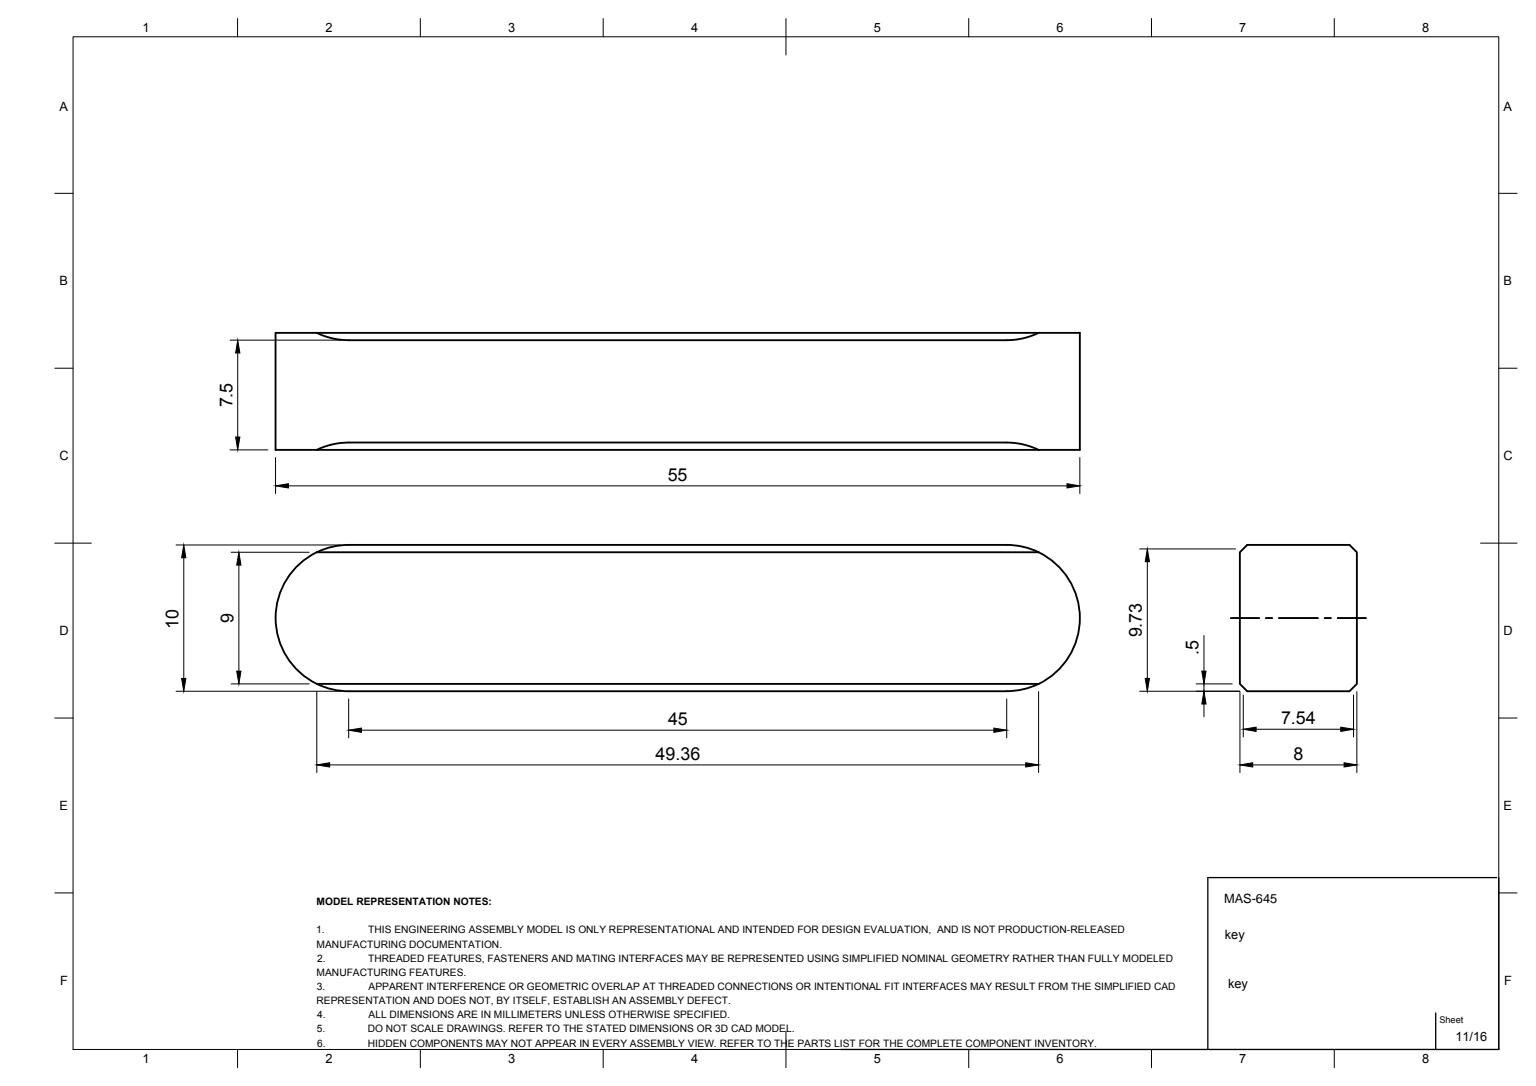
ISO-10303-21;
HEADER;
FILE_DESCRIPTION((''),'2;1');
FILE_NAME('Key.step','2026-10-09T10:54:55-07:00',(''),(''),'','','');
FILE_SCHEMA (('AUTOMOTIVE_DESIGN { 1 0 10303 214 3 1 1 }'));
ENDSEC;
DATA;
#10=MECHANICAL_DESIGN_GEOMETRIC_PRESENTATION_REPRESENTATION('',(#601),#63824);
#91=ELLIPSE('',#16171,7.07106781186547,5.) ;
#92=ELLIPSE('',#16172,7.07106781186548,5.) ;
#93=ELLIPSE('',#16174,7.07106781186548,5.) ;
#94=ELLIPSE('',#16175,7.07106781186547,5.) ;
#95=ELLIPSE('',#16178,7.07106781186546,4.99999999999999) ;
#96=ELLIPSE('',#16180,7.07106781186546,4.99999999999999) ;
#97=ELLIPSE('',#16181,7.07106781186546,4.99999999999999) ;
#98=ELLIPSE('',#16183,7.07106781186546,4.99999999999999) ;
#571=SHAPE_REPRESENTATION_RELATIONSHIP('SRR','None',#63885,#586) ;
#586=ADVANCED_BREP_SHAPE_REPRESENTATION('',(#616),#63815) ;
#601=STYLED_ITEM('',(#63963),#616) ;
#616=MANIFOLD_SOLID_BREP('Body1',#15500) ;
#898=PLANE('',#16176) ;
#899=PLANE('',#16184) ;
#900=PLANE('',#16185) ;
#901=PLANE('',#16186) ;
#902=PLANE('',#16187) ;
#903=PLANE('',#16188) ;
#904=PLANE('',#16189) ;
#905=PLANE('',#16190) ;
#1260=CYLINDRICAL_SURFACE('',#16169,5.) ;
#1261=CYLINDRICAL_SURFACE('',#16177,4.99999999999999) ;
#1815=FACE_OUTER_BOUND('',#2799,.T.) ;
#1816=FACE_OUTER_BOUND('',#2800,.T.) ;
#1817=FACE_OUTER_BOUND('',#2801,.T.) ;
#1818=FACE_OUTER_BOUND('',#2802,.T.) ;
#1819=FACE_OUTER_BOUND('',#2803,.T.) ;
#1820=FACE_OUTER_BOUND('',#2804,.T.) ;
#1821=FACE_OUTER_BOUND('',#2805,.T.) ;
#1822=FACE_OUTER_BOUND('',#2806,.T.) ;
#1823=FACE_OUTER_BOUND('',#2807,.T.) ;
#1824=FACE_OUTER_BOUND('',#2808,.T.) ;
#2799=EDGE_LOOP('',(#10982,#10983,#10984,#10985,#10986,#10987,#10988,#10989)) ;
#2800=EDGE_LOOP('',(#10990,#10991,#10992,#10993)) ;
#2801=EDGE_LOOP('',(#10994,#10995,#10996,#10997,#10998,#10999,#11000,#11001)) ;
#2802=EDGE_LOOP('',(#11002,#11003,#11004,#11005)) ;
#2803=EDGE_LOOP('',(#11006,#11007,#11008,#11009)) ;
#2804=EDGE_LOOP('',(#11010,#11011,#11012,#11013)) ;
#2805=EDGE_LOOP('',(#11014,#11015,#11016,#11017)) ;
#2806=EDGE_LOOP('',(#11018,#11019,#11020,#11021)) ;
#2807=EDGE_LOOP('',(#11022,#11023,#11024,#11025)) ;
#2808=EDGE_LOOP('',(#11026,#11027,#11028,#11029)) ;
#3697=CIRCLE('',#16170,5.) ;
#3698=CIRCLE('',#16173,5.) ;
#3699=CIRCLE('',#16179,4.99999999999999) ;
#3700=CIRCLE('',#16182,4.99999999999999) ;
#4946=LINE('',#51875,#5602) ;
#4947=LINE('',#51883,#5603) ;
#4948=LINE('',#51887,#5604) ;
#4949=LINE('',#51889,#5605) ;
#4950=LINE('',#51890,#5606) ;
#4951=LINE('',#51894,#5607) ;
#4952=LINE('',#51906,#5608) ;
#4953=LINE('',#51907,#5609) ;
#4954=LINE('',#51909,#5610) ;
#4955=LINE('',#51910,#5611) ;
#4956=LINE('',#51912,#5612) ;
#4957=LINE('',#51913,#5613) ;
#5602=VECTOR('',#19152,1000.) ;
#5603=VECTOR('',#19159,1000.) ;
#5604=VECTOR('',#19164,1000.) ;
#5605=VECTOR('',#19165,1000.) ;
#5606=VECTOR('',#19166,1000.) ;
#5607=VECTOR('',#19169,1000.) ;
#5608=VECTOR('',#19184,1000.) ;
#5609=VECTOR('',#19185,1000.) ;
#5610=VECTOR('',#19188,1000.) ;
#5611=VECTOR('',#19189,1000.) ;
#5612=VECTOR('',#19192,1000.) ;
#5613=VECTOR('',#19193,1000.) ;
#6411=VERTEX_POINT('',#51869) ;
#6412=VERTEX_POINT('',#51870) ;
#6413=VERTEX_POINT('',#51872) ;
#6414=VERTEX_POINT('',#51874) ;
#6415=VERTEX_POINT('',#51876) ;
#6416=VERTEX_POINT('',#51878) ;
#6417=VERTEX_POINT('',#51880) ;
#6418=VERTEX_POINT('',#51882) ;
#6419=VERTEX_POINT('',#51886) ;
#6420=VERTEX_POINT('',#51888) ;
#6421=VERTEX_POINT('',#51892) ;
#6422=VERTEX_POINT('',#51893) ;
#6423=VERTEX_POINT('',#51895) ;
#6424=VERTEX_POINT('',#51897) ;
#6425=VERTEX_POINT('',#51900) ;
#6426=VERTEX_POINT('',#51902) ;
#8045=EDGE_CURVE('',#6411,#6412,#3697,.T.) ;
#8046=EDGE_CURVE('',#6412,#6413,#91,.T.) ;
#8047=EDGE_CURVE('',#6414,#6413,#4946,.T.) ;
#8048=EDGE_CURVE('',#6414,#6415,#92,.T.) ;
#8049=EDGE_CURVE('',#6416,#6415,#3698,.T.) ;
#8050=EDGE_CURVE('',#6416,#6417,#93,.T.) ;
#8051=EDGE_CURVE('',#6417,#6418,#4947,.T.) ;
#8052=EDGE_CURVE('',#6418,#6411,#94,.T.) ;
#8053=EDGE_CURVE('',#6419,#6413,#4948,.T.) ;
#8054=EDGE_CURVE('',#6420,#6419,#4949,.T.) ;
#8055=EDGE_CURVE('',#6420,#6414,#4950,.T.) ;
#8056=EDGE_CURVE('',#6421,#6422,#4951,.T.) ;
#8057=EDGE_CURVE('',#6421,#6423,#95,.T.) ;
#8058=EDGE_CURVE('',#6424,#6423,#3699,.T.) ;
#8059=EDGE_CURVE('',#6424,#6420,#96,.T.) ;
#8060=EDGE_CURVE('',#6419,#6425,#97,.T.) ;
#8061=EDGE_CURVE('',#6425,#6426,#3700,.T.) ;
#8062=EDGE_CURVE('',#6426,#6422,#98,.T.) ;
#8063=EDGE_CURVE('',#6421,#6417,#4952,.T.) ;
#8064=EDGE_CURVE('',#6422,#6418,#4953,.T.) ;
#8065=EDGE_CURVE('',#6416,#6423,#4954,.T.) ;
#8066=EDGE_CURVE('',#6424,#6415,#4955,.T.) ;
#8067=EDGE_CURVE('',#6411,#6426,#4956,.T.) ;
#8068=EDGE_CURVE('',#6425,#6412,#4957,.T.) ;
#10982=ORIENTED_EDGE('',*,*,#8045,.T.) ;
#10983=ORIENTED_EDGE('',*,*,#8046,.T.) ;
#10984=ORIENTED_EDGE('',*,*,#8047,.F.) ;
#10985=ORIENTED_EDGE('',*,*,#8048,.T.) ;
#10986=ORIENTED_EDGE('',*,*,#8049,.F.) ;
#10987=ORIENTED_EDGE('',*,*,#8050,.T.) ;
#10988=ORIENTED_EDGE('',*,*,#8051,.T.) ;
#10989=ORIENTED_EDGE('',*,*,#8052,.T.) ;
#10990=ORIENTED_EDGE('',*,*,#8047,.T.) ;
#10991=ORIENTED_EDGE('',*,*,#8053,.F.) ;
#10992=ORIENTED_EDGE('',*,*,#8054,.F.) ;
#10993=ORIENTED_EDGE('',*,*,#8055,.T.) ;
#10994=ORIENTED_EDGE('',*,*,#8056,.F.) ;
#10995=ORIENTED_EDGE('',*,*,#8057,.T.) ;
#10996=ORIENTED_EDGE('',*,*,#8058,.F.) ;
#10997=ORIENTED_EDGE('',*,*,#8059,.T.) ;
#10998=ORIENTED_EDGE('',*,*,#8054,.T.) ;
#10999=ORIENTED_EDGE('',*,*,#8060,.T.) ;
#11000=ORIENTED_EDGE('',*,*,#8061,.T.) ;
#11001=ORIENTED_EDGE('',*,*,#8062,.T.) ;
#11002=ORIENTED_EDGE('',*,*,#8051,.F.) ;
#11003=ORIENTED_EDGE('',*,*,#8063,.F.) ;
#11004=ORIENTED_EDGE('',*,*,#8056,.T.) ;
#11005=ORIENTED_EDGE('',*,*,#8064,.T.) ;
#11006=ORIENTED_EDGE('',*,*,#8065,.F.) ;
#11007=ORIENTED_EDGE('',*,*,#8049,.T.) ;
#11008=ORIENTED_EDGE('',*,*,#8066,.F.) ;
#11009=ORIENTED_EDGE('',*,*,#8058,.T.) ;
#11010=ORIENTED_EDGE('',*,*,#8045,.F.) ;
#11011=ORIENTED_EDGE('',*,*,#8067,.T.) ;
#11012=ORIENTED_EDGE('',*,*,#8061,.F.) ;
#11013=ORIENTED_EDGE('',*,*,#8068,.T.) ;
#11014=ORIENTED_EDGE('',*,*,#8068,.F.) ;
#11015=ORIENTED_EDGE('',*,*,#8060,.F.) ;
#11016=ORIENTED_EDGE('',*,*,#8053,.T.) ;
#11017=ORIENTED_EDGE('',*,*,#8046,.F.) ;
#11018=ORIENTED_EDGE('',*,*,#8064,.F.) ;
#11019=ORIENTED_EDGE('',*,*,#8062,.F.) ;
#11020=ORIENTED_EDGE('',*,*,#8067,.F.) ;
#11021=ORIENTED_EDGE('',*,*,#8052,.F.) ;
#11022=ORIENTED_EDGE('',*,*,#8055,.F.) ;
#11023=ORIENTED_EDGE('',*,*,#8059,.F.) ;
#11024=ORIENTED_EDGE('',*,*,#8066,.T.) ;
#11025=ORIENTED_EDGE('',*,*,#8048,.F.) ;
#11026=ORIENTED_EDGE('',*,*,#8065,.T.) ;
#11027=ORIENTED_EDGE('',*,*,#8057,.F.) ;
#11028=ORIENTED_EDGE('',*,*,#8063,.T.) ;
#11029=ORIENTED_EDGE('',*,*,#8050,.F.) ;
#14903=ADVANCED_FACE('',(#1815),#1260,.T.) ;
#14904=ADVANCED_FACE('',(#1816),#898,.F.) ;
#14905=ADVANCED_FACE('',(#1817),#1261,.T.) ;
#14906=ADVANCED_FACE('',(#1818),#899,.F.) ;
#14907=ADVANCED_FACE('',(#1819),#900,.T.) ;
#14908=ADVANCED_FACE('',(#1820),#901,.F.) ;
#14909=ADVANCED_FACE('',(#1821),#902,.F.) ;
#14910=ADVANCED_FACE('',(#1822),#903,.F.) ;
#14911=ADVANCED_FACE('',(#1823),#904,.F.) ;
#14912=ADVANCED_FACE('',(#1824),#905,.F.) ;
#15500=CLOSED_SHELL('',(#14903,#14904,#14905,#14906,#14907,#14908,#14909,
#14910,#14911,#14912)) ;
#16168=AXIS2_PLACEMENT_3D('',#51867,#19144,#19145) ;
#16169=AXIS2_PLACEMENT_3D('',#51868,#19146,#19147) ;
#16170=AXIS2_PLACEMENT_3D('',#51871,#19148,#19149) ;
#16171=AXIS2_PLACEMENT_3D('',#51873,#19150,#19151) ;
#16172=AXIS2_PLACEMENT_3D('',#51877,#19153,#19154) ;
#16173=AXIS2_PLACEMENT_3D('',#51879,#19155,#19156) ;
#16174=AXIS2_PLACEMENT_3D('',#51881,#19157,#19158) ;
#16175=AXIS2_PLACEMENT_3D('',#51884,#19160,#19161) ;
#16176=AXIS2_PLACEMENT_3D('',#51885,#19162,#19163) ;
#16177=AXIS2_PLACEMENT_3D('',#51891,#19167,#19168) ;
#16178=AXIS2_PLACEMENT_3D('',#51896,#19170,#19171) ;
#16179=AXIS2_PLACEMENT_3D('',#51898,#19172,#19173) ;
#16180=AXIS2_PLACEMENT_3D('',#51899,#19174,#19175) ;
#16181=AXIS2_PLACEMENT_3D('',#51901,#19176,#19177) ;
#16182=AXIS2_PLACEMENT_3D('',#51903,#19178,#19179) ;
#16183=AXIS2_PLACEMENT_3D('',#51904,#19180,#19181) ;
#16184=AXIS2_PLACEMENT_3D('',#51905,#19182,#19183) ;
#16185=AXIS2_PLACEMENT_3D('',#51908,#19186,#19187) ;
#16186=AXIS2_PLACEMENT_3D('',#51911,#19190,#19191) ;
#16187=AXIS2_PLACEMENT_3D('',#51914,#19194,#19195) ;
#16188=AXIS2_PLACEMENT_3D('',#51915,#19196,#19197) ;
#16189=AXIS2_PLACEMENT_3D('',#51916,#19198,#19199) ;
#16190=AXIS2_PLACEMENT_3D('',#51917,#19200,#19201) ;
#19144=DIRECTION('axis',(0.,0.,1.)) ;
#19145=DIRECTION('refdir',(1.,0.,0.)) ;
#19146=DIRECTION('center_axis',(0.,0.,-1.)) ;
#19147=DIRECTION('ref_axis',(-1.,0.,0.)) ;
#19148=DIRECTION('center_axis',(0.,0.,1.)) ;
#19149=DIRECTION('ref_axis',(1.,0.,0.)) ;
#19150=DIRECTION('center_axis',(0.,0.707106781186548,0.707106781186548)) ;
#19151=DIRECTION('ref_axis',(0.,0.707106781186548,-0.707106781186548)) ;
#19152=DIRECTION('',(0.,0.,-1.)) ;
#19153=DIRECTION('center_axis',(0.,0.707106781186548,-0.707106781186547)) ;
#19154=DIRECTION('ref_axis',(0.,-0.707106781186547,-0.707106781186548)) ;
#19155=DIRECTION('center_axis',(0.,0.,1.)) ;
#19156=DIRECTION('ref_axis',(1.,0.,0.)) ;
#19157=DIRECTION('center_axis',(0.,-0.707106781186548,-0.707106781186548)) ;
#19158=DIRECTION('ref_axis',(0.,0.707106781186548,-0.707106781186548)) ;
#19159=DIRECTION('',(0.,0.,-1.)) ;
#19160=DIRECTION('center_axis',(0.,-0.707106781186547,0.707106781186548)) ;
#19161=DIRECTION('ref_axis',(0.,-0.707106781186548,-0.707106781186547)) ;
#19162=DIRECTION('center_axis',(0.,1.,0.)) ;
#19163=DIRECTION('ref_axis',(0.,0.,1.)) ;
#19164=DIRECTION('',(-1.,0.,0.)) ;
#19165=DIRECTION('',(0.,0.,-1.)) ;
#19166=DIRECTION('',(-1.,0.,0.)) ;
#19167=DIRECTION('center_axis',(0.,0.,-1.)) ;
#19168=DIRECTION('ref_axis',(1.,1.22464679914735E-16,0.)) ;
#19169=DIRECTION('',(0.,0.,-1.)) ;
#19170=DIRECTION('center_axis',(0.,-0.707106781186548,-0.707106781186548)) ;
#19171=DIRECTION('ref_axis',(0.,0.707106781186548,-0.707106781186548)) ;
#19172=DIRECTION('center_axis',(0.,0.,1.)) ;
#19173=DIRECTION('ref_axis',(1.,0.,0.)) ;
#19174=DIRECTION('center_axis',(0.,0.707106781186548,-0.707106781186547)) ;
#19175=DIRECTION('ref_axis',(0.,-0.707106781186547,-0.707106781186548)) ;
#19176=DIRECTION('center_axis',(0.,0.707106781186548,0.707106781186548)) ;
#19177=DIRECTION('ref_axis',(0.,0.707106781186548,-0.707106781186548)) ;
#19178=DIRECTION('center_axis',(0.,0.,1.)) ;
#19179=DIRECTION('ref_axis',(1.,0.,0.)) ;
#19180=DIRECTION('center_axis',(0.,-0.707106781186547,0.707106781186548)) ;
#19181=DIRECTION('ref_axis',(0.,-0.707106781186548,-0.707106781186547)) ;
#19182=DIRECTION('center_axis',(0.,-1.,0.)) ;
#19183=DIRECTION('ref_axis',(0.,0.,-1.)) ;
#19184=DIRECTION('',(-1.,0.,0.)) ;
#19185=DIRECTION('',(-1.,0.,0.)) ;
#19186=DIRECTION('center_axis',(0.,0.,1.)) ;
#19187=DIRECTION('ref_axis',(1.,0.,0.)) ;
#19188=DIRECTION('',(1.,0.,0.)) ;
#19189=DIRECTION('',(-1.,0.,0.)) ;
#19190=DIRECTION('center_axis',(0.,0.,1.)) ;
#19191=DIRECTION('ref_axis',(1.,0.,0.)) ;
#19192=DIRECTION('',(1.,0.,0.)) ;
#19193=DIRECTION('',(-1.,0.,0.)) ;
#19194=DIRECTION('center_axis',(0.,0.707106781186548,0.707106781186548)) ;
#19195=DIRECTION('ref_axis',(0.,-0.707106781186548,0.707106781186548)) ;
#19196=DIRECTION('center_axis',(0.,-0.707106781186547,0.707106781186548)) ;
#19197=DIRECTION('ref_axis',(0.,-0.707106781186548,-0.707106781186547)) ;
#19198=DIRECTION('center_axis',(0.,0.707106781186548,-0.707106781186547)) ;
#19199=DIRECTION('ref_axis',(0.,0.707106781186547,0.707106781186548)) ;
#19200=DIRECTION('center_axis',(0.,-0.707106781186548,-0.707106781186548)) ;
#19201=DIRECTION('ref_axis',(0.,0.707106781186548,-0.707106781186548)) ;
#51867=CARTESIAN_POINT('',(0.,0.,0.)) ;
#51868=CARTESIAN_POINT('Origin',(5.,5.,8.)) ;
#51869=CARTESIAN_POINT('',(2.82055052822966,9.5,0.)) ;
#51870=CARTESIAN_POINT('',(2.82055052822966,0.5,0.)) ;
#51871=CARTESIAN_POINT('Origin',(5.,5.,0.)) ;
#51872=CARTESIAN_POINT('',(5.,0.,0.500000000000001)) ;
#51873=CARTESIAN_POINT('Origin',(5.,5.,-4.5)) ;
#51874=CARTESIAN_POINT('',(5.,0.,7.5)) ;
#51875=CARTESIAN_POINT('',(5.,-8.67361737988404E-16,8.)) ;
#51876=CARTESIAN_POINT('',(2.82055052822966,0.5,8.)) ;
#51877=CARTESIAN_POINT('Origin',(5.,5.,12.5)) ;
#51878=CARTESIAN_POINT('',(2.82055052822966,9.5,8.)) ;
#51879=CARTESIAN_POINT('Origin',(5.,5.,8.)) ;
#51880=CARTESIAN_POINT('',(5.,10.,7.5)) ;
#51881=CARTESIAN_POINT('Origin',(5.,5.,12.5)) ;
#51882=CARTESIAN_POINT('',(5.,10.,0.5)) ;
#51883=CARTESIAN_POINT('',(5.,10.,8.)) ;
#51884=CARTESIAN_POINT('Origin',(5.,5.,-4.5)) ;
#51885=CARTESIAN_POINT('Origin',(5.,0.,8.)) ;
#51886=CARTESIAN_POINT('',(50.,0.,0.500000000000001)) ;
#51887=CARTESIAN_POINT('',(55.,0.,0.500000000000001)) ;
#51888=CARTESIAN_POINT('',(50.,8.67361737988404E-16,7.5)) ;
#51889=CARTESIAN_POINT('',(50.,0.,8.)) ;
#51890=CARTESIAN_POINT('',(55.,0.,7.5)) ;
#51891=CARTESIAN_POINT('Origin',(50.,5.00000000000001,8.)) ;
#51892=CARTESIAN_POINT('',(50.,10.,7.5)) ;
#51893=CARTESIAN_POINT('',(50.,10.,0.5)) ;
#51894=CARTESIAN_POINT('',(50.,10.,8.)) ;
#51895=CARTESIAN_POINT('',(52.1794494717703,9.5,8.)) ;
#51896=CARTESIAN_POINT('Origin',(50.,5.00000000000001,12.5)) ;
#51897=CARTESIAN_POINT('',(52.1794494717703,0.5,8.)) ;
#51898=CARTESIAN_POINT('Origin',(50.,5.00000000000001,8.)) ;
#51899=CARTESIAN_POINT('Origin',(50.,4.99999999999999,12.5)) ;
#51900=CARTESIAN_POINT('',(52.1794494717703,0.5,0.)) ;
#51901=CARTESIAN_POINT('Origin',(50.,4.99999999999999,-4.49999999999999)) ;
#51902=CARTESIAN_POINT('',(52.1794494717703,9.5,0.)) ;
#51903=CARTESIAN_POINT('Origin',(50.,5.00000000000001,0.)) ;
#51904=CARTESIAN_POINT('Origin',(50.,5.00000000000001,-4.49999999999998)) ;
#51905=CARTESIAN_POINT('Origin',(50.,10.,8.)) ;
#51906=CARTESIAN_POINT('',(55.,10.,7.5)) ;
#51907=CARTESIAN_POINT('',(55.,10.,0.5)) ;
#51908=CARTESIAN_POINT('Origin',(5.,5.,8.)) ;
#51909=CARTESIAN_POINT('',(5.,9.5,8.)) ;
#51910=CARTESIAN_POINT('',(5.,0.5,8.)) ;
#51911=CARTESIAN_POINT('Origin',(5.,5.,0.)) ;
#51912=CARTESIAN_POINT('',(5.,9.5,0.)) ;
#51913=CARTESIAN_POINT('',(5.,0.5,0.)) ;
#51914=CARTESIAN_POINT('Origin',(55.,0.,0.5)) ;
#51915=CARTESIAN_POINT('Origin',(55.,9.5,0.)) ;
#51916=CARTESIAN_POINT('Origin',(55.,0.5,8.)) ;
#51917=CARTESIAN_POINT('Origin',(55.,10.,7.5)) ;
#63798=UNCERTAINTY_MEASURE_WITH_UNIT(LENGTH_MEASURE(0.01),#63825,
'DISTANCE_ACCURACY_VALUE',
'Maximum model space distance between geometric entities at asserted c
onnectivities') ;
#63807=UNCERTAINTY_MEASURE_WITH_UNIT(LENGTH_MEASURE(0.01),#63825,
'DISTANCE_ACCURACY_VALUE',
'Maximum model space distance between geometric entities at asserted c
onnectivities') ;
#63815=(
GEOMETRIC_REPRESENTATION_CONTEXT(3)
GLOBAL_UNCERTAINTY_ASSIGNED_CONTEXT((#63798))
GLOBAL_UNIT_ASSIGNED_CONTEXT((#63825,#63827,#63828))
REPRESENTATION_CONTEXT('','3D')
) ;
#63824=(
GEOMETRIC_REPRESENTATION_CONTEXT(3)
GLOBAL_UNCERTAINTY_ASSIGNED_CONTEXT((#63807))
GLOBAL_UNIT_ASSIGNED_CONTEXT((#63825,#63827,#63828))
REPRESENTATION_CONTEXT('','3D')
) ;
#63825=(
LENGTH_UNIT()
NAMED_UNIT(*)
SI_UNIT(.MILLI.,.METRE.)
) ;
#63827=(
NAMED_UNIT(*)
PLANE_ANGLE_UNIT()
SI_UNIT($,.RADIAN.)
) ;
#63828=(
NAMED_UNIT(*)
SI_UNIT($,.STERADIAN.)
SOLID_ANGLE_UNIT()
) ;
#63836=SHAPE_DEFINITION_REPRESENTATION(#63852,#63885) ;
#63852=PRODUCT_DEFINITION_SHAPE('',$,#63902) ;
#63885=SHAPE_REPRESENTATION('',(#16168),#63815) ;
#63894=PRODUCT_DEFINITION_CONTEXT('part definition',#63944,'design') ;
#63902=PRODUCT_DEFINITION('Key','Key',#63918,#63894) ;
#63918=PRODUCT_DEFINITION_FORMATION('',$,#63953) ;
#63944=APPLICATION_CONTEXT(
'Core Data for Automotive Mechanical Design Process') ;
#63945=PRODUCT_CONTEXT('part definition',#63944,'mechanical') ;
#63953=PRODUCT('Key','Key',$,(#63945)) ;
#63963=PRESENTATION_STYLE_ASSIGNMENT((#63968)) ;
#63968=SURFACE_STYLE_USAGE(.BOTH.,#63973) ;
#63973=SURFACE_SIDE_STYLE('',(#63978)) ;
#63978=SURFACE_STYLE_FILL_AREA(#63983) ;
#63983=FILL_AREA_STYLE('Opaque(160,160,160)',(#63988)) ;
#63988=FILL_AREA_STYLE_COLOUR('Opaque(160,160,160)',#63993) ;
#63993=COLOUR_RGB('Opaque(160,160,160)', 0.09019608, 0.27058824, 0.51372549) ;
ENDSEC;
END-ISO-10303-21;
